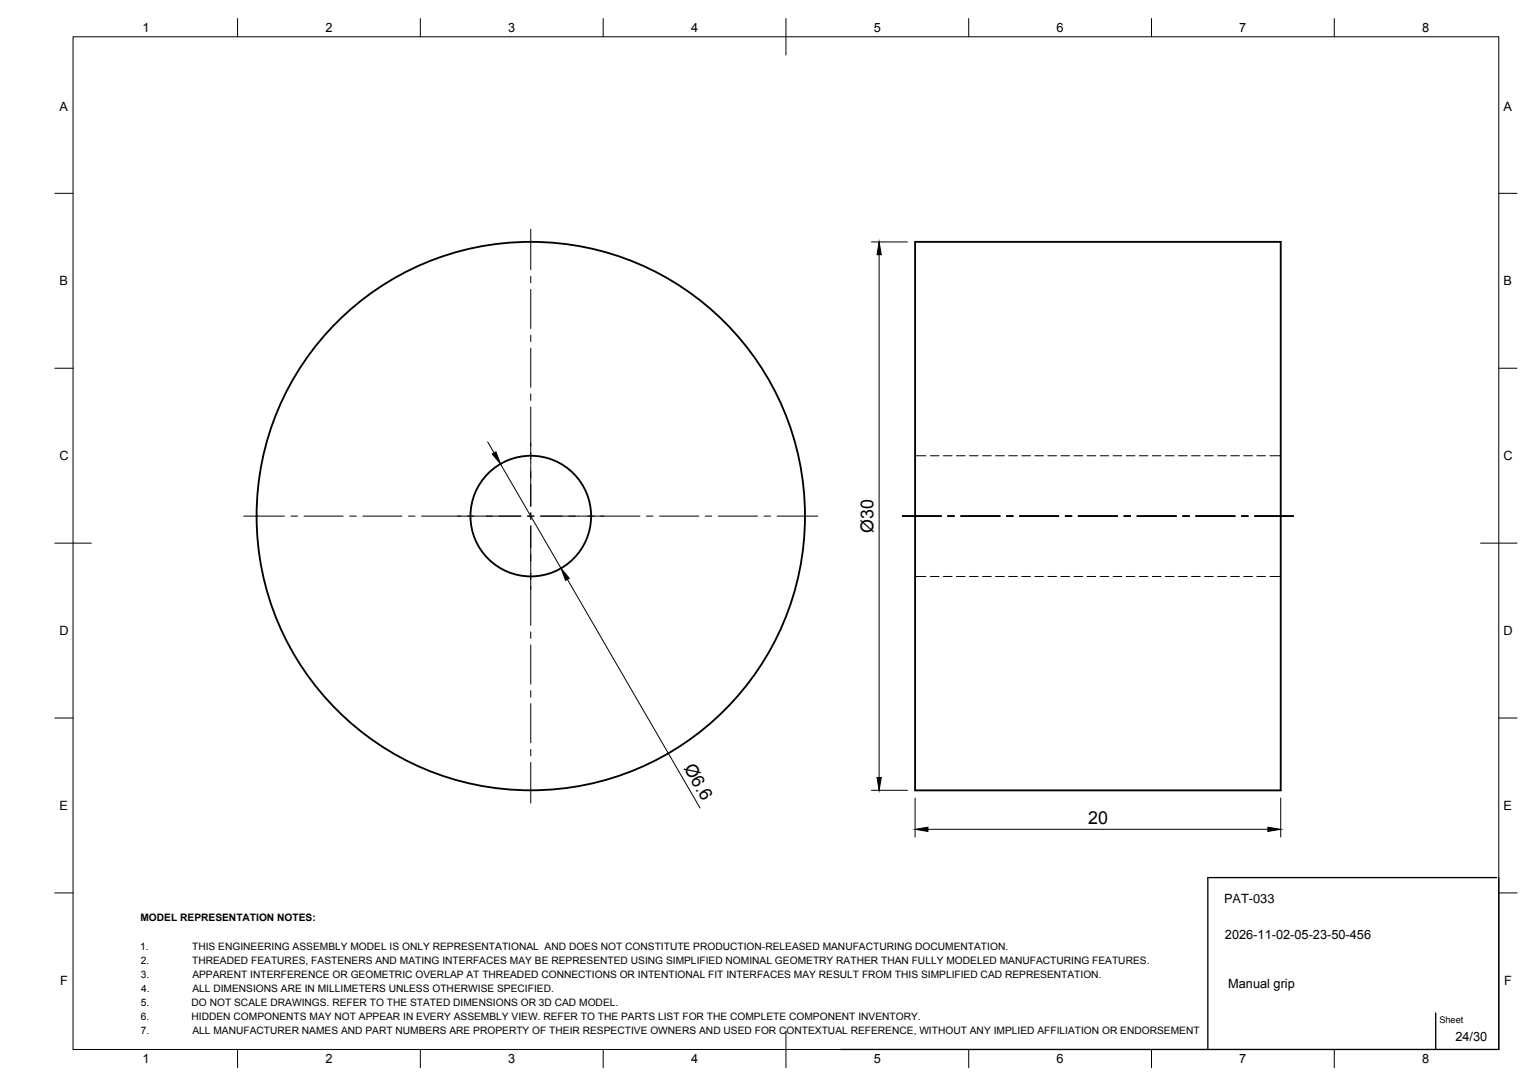
ISO-10303-21;
HEADER;
/* Generated by software containing ST-Developer
 * from STEP Tools, Inc. (www.steptools.com) 
 */

FILE_DESCRIPTION(
/* description */ ('Dual-rail gantry carriage'),
/* implementation_level */ '2;1');

FILE_NAME(
/* name */ 'Manual grip.step',
/* time_stamp */ '2026-10-27T10:49:15-07:00',
/* author */ (''),
/* organization */ (''),
/* preprocessor_version */ 'ST-DEVELOPER v20.2',
/* originating_system */ 'Autodesk Translation Framework v15.17.0.0',
/* authorisation */ '');

FILE_SCHEMA (('AUTOMOTIVE_DESIGN { 1 0 10303 214 3 1 1 }'));
ENDSEC;

DATA;
#10=MECHANICAL_DESIGN_GEOMETRIC_PRESENTATION_REPRESENTATION('',(#605),#12804);
#543=SHAPE_REPRESENTATION_RELATIONSHIP('SRR','None',#13022,#574);
#574=ADVANCED_BREP_SHAPE_REPRESENTATION('',(#634),#12792);
#605=STYLED_ITEM('',(#13254),#634);
#634=MANIFOLD_SOLID_BREP('Body1',#7385);
#745=FACE_BOUND('',#1812,.T.);
#746=FACE_BOUND('',#1814,.T.);
#961=PLANE('',#8181);
#962=PLANE('',#8182);
#1317=FACE_OUTER_BOUND('',#1809,.T.);
#1318=FACE_OUTER_BOUND('',#1810,.T.);
#1319=FACE_OUTER_BOUND('',#1811,.T.);
#1320=FACE_OUTER_BOUND('',#1813,.T.);
#1809=EDGE_LOOP('',(#6357,#6358,#6359,#6360));
#1810=EDGE_LOOP('',(#6361,#6362,#6363,#6364));
#1811=EDGE_LOOP('',(#6365));
#1812=EDGE_LOOP('',(#6366));
#1813=EDGE_LOOP('',(#6367));
#1814=EDGE_LOOP('',(#6368));
#2452=LINE('',#12047,#3161);
#2453=LINE('',#12053,#3162);
#3161=VECTOR('',#9863,0.329999999999998);
#3162=VECTOR('',#9870,1.5);
#3505=CIRCLE('',#8176,0.329999999999998);
#3506=CIRCLE('',#8177,0.329999999999998);
#3507=CIRCLE('',#8179,1.5);
#3508=CIRCLE('',#8180,1.5);
#3983=VERTEX_POINT('',#12044);
#3984=VERTEX_POINT('',#12046);
#3985=VERTEX_POINT('',#12050);
#3986=VERTEX_POINT('',#12052);
#4801=EDGE_CURVE('',#3983,#3983,#3505,.T.);
#4802=EDGE_CURVE('',#3983,#3984,#2452,.T.);
#4803=EDGE_CURVE('',#3984,#3984,#3506,.T.);
#4804=EDGE_CURVE('',#3985,#3985,#3507,.T.);
#4805=EDGE_CURVE('',#3985,#3986,#2453,.T.);
#4806=EDGE_CURVE('',#3986,#3986,#3508,.T.);
#6357=ORIENTED_EDGE('',*,*,#4801,.F.);
#6358=ORIENTED_EDGE('',*,*,#4802,.T.);
#6359=ORIENTED_EDGE('',*,*,#4803,.T.);
#6360=ORIENTED_EDGE('',*,*,#4802,.F.);
#6361=ORIENTED_EDGE('',*,*,#4804,.F.);
#6362=ORIENTED_EDGE('',*,*,#4805,.T.);
#6363=ORIENTED_EDGE('',*,*,#4806,.T.);
#6364=ORIENTED_EDGE('',*,*,#4805,.F.);
#6365=ORIENTED_EDGE('',*,*,#4804,.T.);
#6366=ORIENTED_EDGE('',*,*,#4801,.T.);
#6367=ORIENTED_EDGE('',*,*,#4806,.F.);
#6368=ORIENTED_EDGE('',*,*,#4803,.F.);
#6954=CYLINDRICAL_SURFACE('',#8175,0.329999999999998);
#6955=CYLINDRICAL_SURFACE('',#8178,1.5);
#7243=ADVANCED_FACE('',(#1317),#6954,.F.);
#7244=ADVANCED_FACE('',(#1318),#6955,.T.);
#7245=ADVANCED_FACE('',(#1319,#745),#961,.T.);
#7246=ADVANCED_FACE('',(#1320,#746),#962,.F.);
#7385=CLOSED_SHELL('',(#7243,#7244,#7245,#7246));
#8174=AXIS2_PLACEMENT_3D('',#12042,#9857,#9858);
#8175=AXIS2_PLACEMENT_3D('',#12043,#9859,#9860);
#8176=AXIS2_PLACEMENT_3D('',#12045,#9861,#9862);
#8177=AXIS2_PLACEMENT_3D('',#12048,#9864,#9865);
#8178=AXIS2_PLACEMENT_3D('',#12049,#9866,#9867);
#8179=AXIS2_PLACEMENT_3D('',#12051,#9868,#9869);
#8180=AXIS2_PLACEMENT_3D('',#12054,#9871,#9872);
#8181=AXIS2_PLACEMENT_3D('',#12055,#9873,#9874);
#8182=AXIS2_PLACEMENT_3D('',#12056,#9875,#9876);
#9857=DIRECTION('axis',(0.,0.,1.));
#9858=DIRECTION('refdir',(1.,0.,0.));
#9859=DIRECTION('center_axis',(0.,0.,1.));
#9860=DIRECTION('ref_axis',(1.,0.,0.));
#9861=DIRECTION('center_axis',(0.,0.,-1.));
#9862=DIRECTION('ref_axis',(1.,0.,0.));
#9863=DIRECTION('',(0.,0.,-1.));
#9864=DIRECTION('center_axis',(0.,0.,-1.));
#9865=DIRECTION('ref_axis',(1.,0.,0.));
#9866=DIRECTION('center_axis',(0.,0.,1.));
#9867=DIRECTION('ref_axis',(1.,0.,0.));
#9868=DIRECTION('center_axis',(0.,0.,1.));
#9869=DIRECTION('ref_axis',(1.,0.,0.));
#9870=DIRECTION('',(0.,0.,-1.));
#9871=DIRECTION('center_axis',(0.,0.,1.));
#9872=DIRECTION('ref_axis',(1.,0.,0.));
#9873=DIRECTION('center_axis',(0.,0.,1.));
#9874=DIRECTION('ref_axis',(1.,0.,0.));
#9875=DIRECTION('center_axis',(0.,0.,1.));
#9876=DIRECTION('ref_axis',(1.,0.,0.));
#12042=CARTESIAN_POINT('',(0.,0.,0.));
#12043=CARTESIAN_POINT('Origin',(20.,0.,6.4));
#12044=CARTESIAN_POINT('',(19.67,-4.04133443718624E-17,8.4));
#12045=CARTESIAN_POINT('Origin',(20.,0.,8.4));
#12046=CARTESIAN_POINT('',(19.67,-4.04133443718624E-17,6.4));
#12047=CARTESIAN_POINT('',(19.67,-4.04133443718624E-17,6.4));
#12048=CARTESIAN_POINT('Origin',(20.,0.,6.4));
#12049=CARTESIAN_POINT('Origin',(20.,0.,6.4));
#12050=CARTESIAN_POINT('',(18.5,-1.83697019872103E-16,8.4));
#12051=CARTESIAN_POINT('Origin',(20.,0.,8.4));
#12052=CARTESIAN_POINT('',(18.5,-1.83697019872103E-16,6.4));
#12053=CARTESIAN_POINT('',(18.5,-1.83697019872103E-16,6.4));
#12054=CARTESIAN_POINT('Origin',(20.,0.,6.4));
#12055=CARTESIAN_POINT('Origin',(20.,0.,8.4));
#12056=CARTESIAN_POINT('Origin',(20.,0.,6.4));
#12756=UNCERTAINTY_MEASURE_WITH_UNIT(LENGTH_MEASURE(0.001),#12805,
'DISTANCE_ACCURACY_VALUE',
'Maximum model space distance between geometric entities at asserted c
onnectivities');
#12768=UNCERTAINTY_MEASURE_WITH_UNIT(LENGTH_MEASURE(0.001),#12805,
'DISTANCE_ACCURACY_VALUE',
'Maximum model space distance between geometric entities at asserted c
onnectivities');
#12792=(
GEOMETRIC_REPRESENTATION_CONTEXT(3)
GLOBAL_UNCERTAINTY_ASSIGNED_CONTEXT((#12756))
GLOBAL_UNIT_ASSIGNED_CONTEXT((#12805,#12807,#12808))
REPRESENTATION_CONTEXT('','3D')
);
#12804=(
GEOMETRIC_REPRESENTATION_CONTEXT(3)
GLOBAL_UNCERTAINTY_ASSIGNED_CONTEXT((#12768))
GLOBAL_UNIT_ASSIGNED_CONTEXT((#12805,#12807,#12808))
REPRESENTATION_CONTEXT('','3D')
);
#12805=(
LENGTH_UNIT()
NAMED_UNIT(*)
SI_UNIT(.CENTI.,.METRE.)
);
#12807=(
NAMED_UNIT(*)
PLANE_ANGLE_UNIT()
SI_UNIT($,.RADIAN.)
);
#12808=(
NAMED_UNIT(*)
SI_UNIT($,.STERADIAN.)
SOLID_ANGLE_UNIT()
);
#12832=SHAPE_DEFINITION_REPRESENTATION(#12867,#13022);
#12867=PRODUCT_DEFINITION_SHAPE('',$,#13058);
#13022=SHAPE_REPRESENTATION('',(#8174),#12792);
#13034=PRODUCT_DEFINITION_CONTEXT('part definition',#13141,'design');
#13058=PRODUCT_DEFINITION('Manual grip','Manual grip',#13093,#13034);
#13093=PRODUCT_DEFINITION_FORMATION('',$,#13166);
#13141=APPLICATION_CONTEXT(
'Core Data for Automotive Mechanical Design Process');
#13142=PRODUCT_CONTEXT('part definition',#13141,'mechanical');
#13166=PRODUCT('Manual grip','Manual grip','Manual grip',(#13142));
#13248=COLOUR_RGB('Black',0.12,0.14,0.17);
#13249=FILL_AREA_STYLE_COLOUR('',#13248);
#13250=FILL_AREA_STYLE('',(#13249));
#13251=SURFACE_STYLE_FILL_AREA(#13250);
#13252=SURFACE_SIDE_STYLE('',(#13251));
#13253=SURFACE_STYLE_USAGE(.BOTH.,#13252);
#13254=PRESENTATION_STYLE_ASSIGNMENT((#13253));
ENDSEC;
END-ISO-10303-21;
